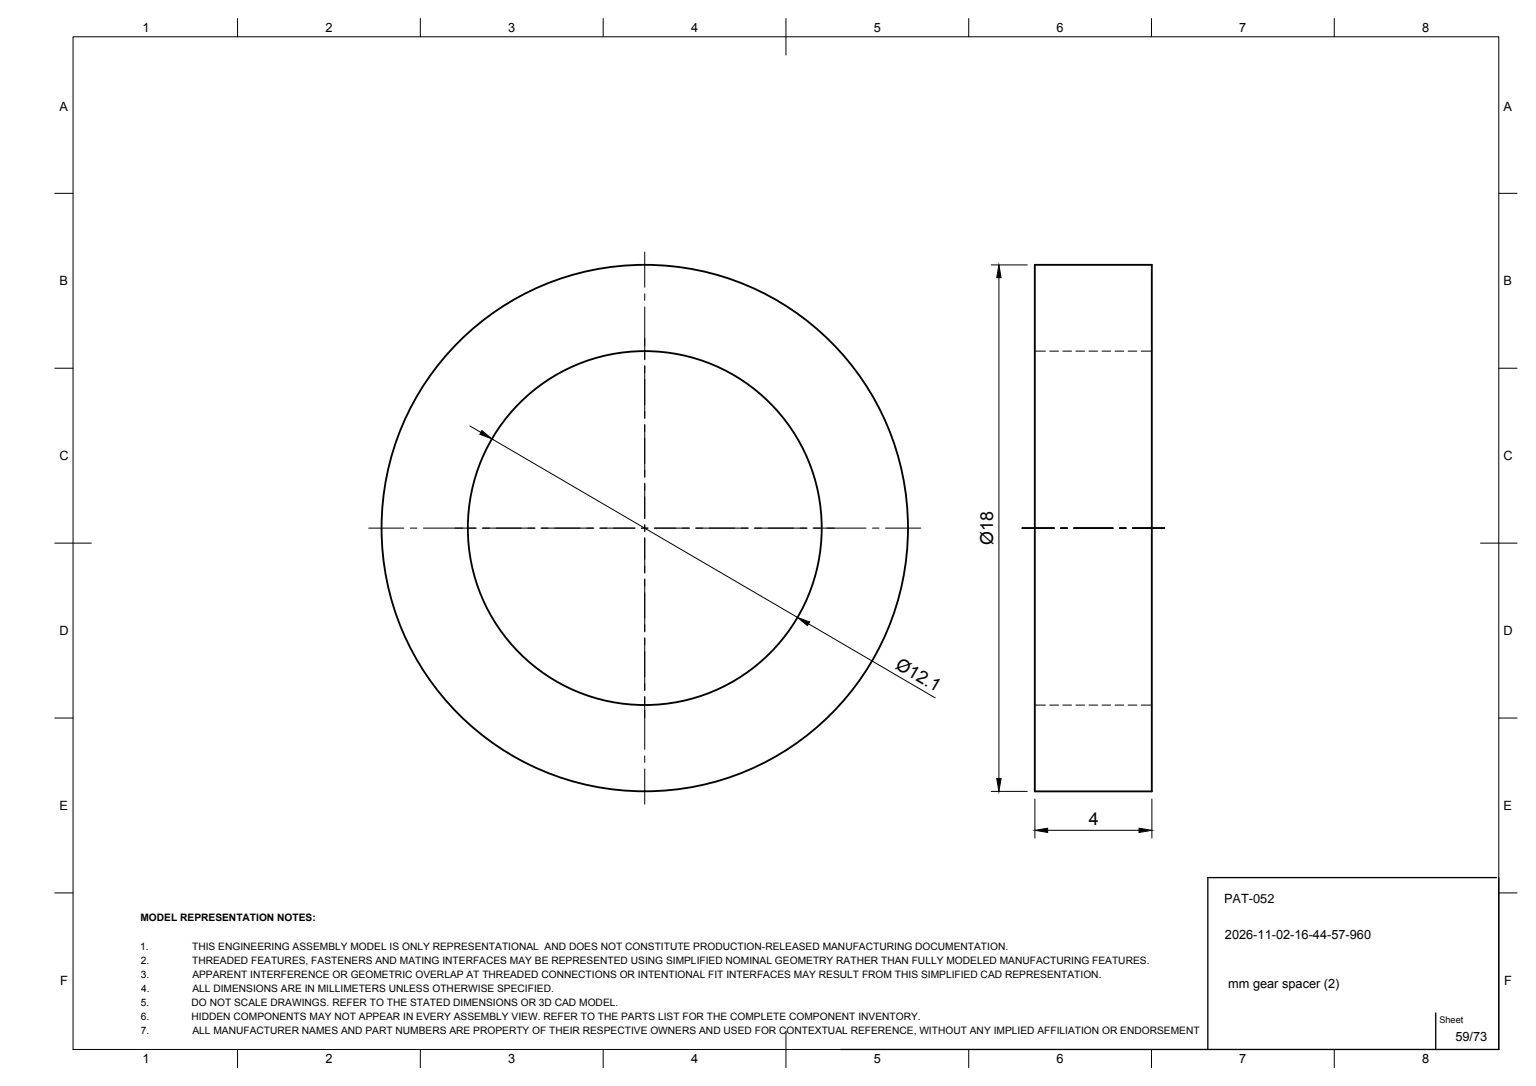
ISO-10303-21;
HEADER;
/* Generated by software containing ST-Developer
 * from STEP Tools, Inc. (www.steptools.com) 
 */

FILE_DESCRIPTION(
/* description */ ('Hand-crank gear train demonstrator'),
/* implementation_level */ '2;1');

FILE_NAME(
/* name */ 'mm gear spacer (2).step',
/* time_stamp */ '2026-10-28T03:22:13-07:00',
/* author */ (''),
/* organization */ (''),
/* preprocessor_version */ 'ST-DEVELOPER v20.2',
/* originating_system */ 'Autodesk Translation Framework v15.17.0.0',
/* authorisation */ '');

FILE_SCHEMA (('AUTOMOTIVE_DESIGN { 1 0 10303 214 3 1 1 }'));
ENDSEC;

DATA;
#10=MECHANICAL_DESIGN_GEOMETRIC_PRESENTATION_REPRESENTATION('',(#1249),#62758);
#1106=SHAPE_REPRESENTATION_RELATIONSHIP('SRR','None',#63083,#1170);
#1170=ADVANCED_BREP_SHAPE_REPRESENTATION('',(#1324),#62737);
#1249=STYLED_ITEM('',(#63476),#1324);
#1324=MANIFOLD_SOLID_BREP('Body1',#16433);
#1590=FACE_BOUND('',#3866,.T.);
#1591=FACE_BOUND('',#3868,.T.);
#1967=PLANE('',#18236);
#1968=PLANE('',#18237);
#2679=FACE_OUTER_BOUND('',#3863,.T.);
#2680=FACE_OUTER_BOUND('',#3864,.T.);
#2681=FACE_OUTER_BOUND('',#3865,.T.);
#2682=FACE_OUTER_BOUND('',#3867,.T.);
#3863=EDGE_LOOP('',(#13187,#13188,#13189,#13190));
#3864=EDGE_LOOP('',(#13191,#13192,#13193,#13194));
#3865=EDGE_LOOP('',(#13195));
#3866=EDGE_LOOP('',(#13196));
#3867=EDGE_LOOP('',(#13197));
#3868=EDGE_LOOP('',(#13198));
#4969=LINE('',#26650,#6101);
#4970=LINE('',#26656,#6102);
#6101=VECTOR('',#21662,0.605);
#6102=VECTOR('',#21669,0.9);
#7003=CIRCLE('',#18231,0.605);
#7004=CIRCLE('',#18232,0.605);
#7005=CIRCLE('',#18234,0.9);
#7006=CIRCLE('',#18235,0.9);
#8010=VERTEX_POINT('',#26647);
#8011=VERTEX_POINT('',#26649);
#8012=VERTEX_POINT('',#26653);
#8013=VERTEX_POINT('',#26655);
#9845=EDGE_CURVE('',#8010,#8010,#7003,.T.);
#9846=EDGE_CURVE('',#8010,#8011,#4969,.T.);
#9847=EDGE_CURVE('',#8011,#8011,#7004,.T.);
#9848=EDGE_CURVE('',#8012,#8012,#7005,.T.);
#9849=EDGE_CURVE('',#8012,#8013,#4970,.T.);
#9850=EDGE_CURVE('',#8013,#8013,#7006,.T.);
#13187=ORIENTED_EDGE('',*,*,#9845,.F.);
#13188=ORIENTED_EDGE('',*,*,#9846,.T.);
#13189=ORIENTED_EDGE('',*,*,#9847,.T.);
#13190=ORIENTED_EDGE('',*,*,#9846,.F.);
#13191=ORIENTED_EDGE('',*,*,#9848,.F.);
#13192=ORIENTED_EDGE('',*,*,#9849,.T.);
#13193=ORIENTED_EDGE('',*,*,#9850,.T.);
#13194=ORIENTED_EDGE('',*,*,#9849,.F.);
#13195=ORIENTED_EDGE('',*,*,#9848,.T.);
#13196=ORIENTED_EDGE('',*,*,#9845,.T.);
#13197=ORIENTED_EDGE('',*,*,#9850,.F.);
#13198=ORIENTED_EDGE('',*,*,#9847,.F.);
#15335=CYLINDRICAL_SURFACE('',#18230,0.605);
#15336=CYLINDRICAL_SURFACE('',#18233,0.9);
#15989=ADVANCED_FACE('',(#2679),#15335,.F.);
#15990=ADVANCED_FACE('',(#2680),#15336,.T.);
#15991=ADVANCED_FACE('',(#2681,#1590),#1967,.T.);
#15992=ADVANCED_FACE('',(#2682,#1591),#1968,.F.);
#16433=CLOSED_SHELL('',(#15989,#15990,#15991,#15992));
#18229=AXIS2_PLACEMENT_3D('',#26645,#21656,#21657);
#18230=AXIS2_PLACEMENT_3D('',#26646,#21658,#21659);
#18231=AXIS2_PLACEMENT_3D('',#26648,#21660,#21661);
#18232=AXIS2_PLACEMENT_3D('',#26651,#21663,#21664);
#18233=AXIS2_PLACEMENT_3D('',#26652,#21665,#21666);
#18234=AXIS2_PLACEMENT_3D('',#26654,#21667,#21668);
#18235=AXIS2_PLACEMENT_3D('',#26657,#21670,#21671);
#18236=AXIS2_PLACEMENT_3D('',#26658,#21672,#21673);
#18237=AXIS2_PLACEMENT_3D('',#26659,#21674,#21675);
#21656=DIRECTION('axis',(0.,0.,1.));
#21657=DIRECTION('refdir',(1.,0.,0.));
#21658=DIRECTION('center_axis',(0.,1.,0.));
#21659=DIRECTION('ref_axis',(1.,0.,0.));
#21660=DIRECTION('center_axis',(0.,-1.,0.));
#21661=DIRECTION('ref_axis',(1.,0.,0.));
#21662=DIRECTION('',(0.,-1.,0.));
#21663=DIRECTION('center_axis',(0.,-1.,0.));
#21664=DIRECTION('ref_axis',(1.,0.,0.));
#21665=DIRECTION('center_axis',(0.,1.,0.));
#21666=DIRECTION('ref_axis',(1.,0.,0.));
#21667=DIRECTION('center_axis',(0.,1.,0.));
#21668=DIRECTION('ref_axis',(1.,0.,0.));
#21669=DIRECTION('',(0.,-1.,0.));
#21670=DIRECTION('center_axis',(0.,1.,0.));
#21671=DIRECTION('ref_axis',(1.,0.,0.));
#21672=DIRECTION('center_axis',(0.,1.,0.));
#21673=DIRECTION('ref_axis',(1.,0.,0.));
#21674=DIRECTION('center_axis',(0.,1.,0.));
#21675=DIRECTION('ref_axis',(1.,0.,0.));
#26645=CARTESIAN_POINT('',(0.,0.,0.));
#26646=CARTESIAN_POINT('Origin',(12.,-0.4,9.));
#26647=CARTESIAN_POINT('',(11.395,0.,9.));
#26648=CARTESIAN_POINT('Origin',(12.,0.,9.));
#26649=CARTESIAN_POINT('',(11.395,-0.4,9.));
#26650=CARTESIAN_POINT('',(11.395,-0.4,9.));
#26651=CARTESIAN_POINT('Origin',(12.,-0.4,9.));
#26652=CARTESIAN_POINT('Origin',(12.,-0.4,9.));
#26653=CARTESIAN_POINT('',(11.1,0.,9.));
#26654=CARTESIAN_POINT('Origin',(12.,0.,9.));
#26655=CARTESIAN_POINT('',(11.1,-0.4,9.));
#26656=CARTESIAN_POINT('',(11.1,-0.4,9.));
#26657=CARTESIAN_POINT('Origin',(12.,-0.4,9.));
#26658=CARTESIAN_POINT('Origin',(12.,0.,9.));
#26659=CARTESIAN_POINT('Origin',(12.,-0.4,9.));
#62663=UNCERTAINTY_MEASURE_WITH_UNIT(LENGTH_MEASURE(0.001),#62759,
'DISTANCE_ACCURACY_VALUE',
'Maximum model space distance between geometric entities at asserted c
onnectivities');
#62684=UNCERTAINTY_MEASURE_WITH_UNIT(LENGTH_MEASURE(0.001),#62759,
'DISTANCE_ACCURACY_VALUE',
'Maximum model space distance between geometric entities at asserted c
onnectivities');
#62737=(
GEOMETRIC_REPRESENTATION_CONTEXT(3)
GLOBAL_UNCERTAINTY_ASSIGNED_CONTEXT((#62663))
GLOBAL_UNIT_ASSIGNED_CONTEXT((#62759,#62761,#62762))
REPRESENTATION_CONTEXT('','3D')
);
#62758=(
GEOMETRIC_REPRESENTATION_CONTEXT(3)
GLOBAL_UNCERTAINTY_ASSIGNED_CONTEXT((#62684))
GLOBAL_UNIT_ASSIGNED_CONTEXT((#62759,#62761,#62762))
REPRESENTATION_CONTEXT('','3D')
);
#62759=(
LENGTH_UNIT()
NAMED_UNIT(*)
SI_UNIT(.CENTI.,.METRE.)
);
#62761=(
NAMED_UNIT(*)
PLANE_ANGLE_UNIT()
SI_UNIT($,.RADIAN.)
);
#62762=(
NAMED_UNIT(*)
SI_UNIT($,.STERADIAN.)
SOLID_ANGLE_UNIT()
);
#62815=SHAPE_DEFINITION_REPRESENTATION(#62898,#63083);
#62898=PRODUCT_DEFINITION_SHAPE('',$,#63157);
#63083=SHAPE_REPRESENTATION('',(#18229),#62737);
#63104=PRODUCT_DEFINITION_CONTEXT('part definition',#63325,'design');
#63157=PRODUCT_DEFINITION('mm gear spacer (2)','mm gear spacer (2)',#63230,
#63104);
#63230=PRODUCT_DEFINITION_FORMATION('',$,#63379);
#63325=APPLICATION_CONTEXT(
'Core Data for Automotive Mechanical Design Process');
#63326=PRODUCT_CONTEXT('part definition',#63325,'mechanical');
#63379=PRODUCT('mm gear spacer (2)','mm gear spacer (2)','mm gear spacer (2)',
(#63326));
#63470=COLOUR_RGB('Off White',0.89,0.88,0.83);
#63471=FILL_AREA_STYLE_COLOUR('',#63470);
#63472=FILL_AREA_STYLE('',(#63471));
#63473=SURFACE_STYLE_FILL_AREA(#63472);
#63474=SURFACE_SIDE_STYLE('',(#63473));
#63475=SURFACE_STYLE_USAGE(.BOTH.,#63474);
#63476=PRESENTATION_STYLE_ASSIGNMENT((#63475));
ENDSEC;
END-ISO-10303-21;
